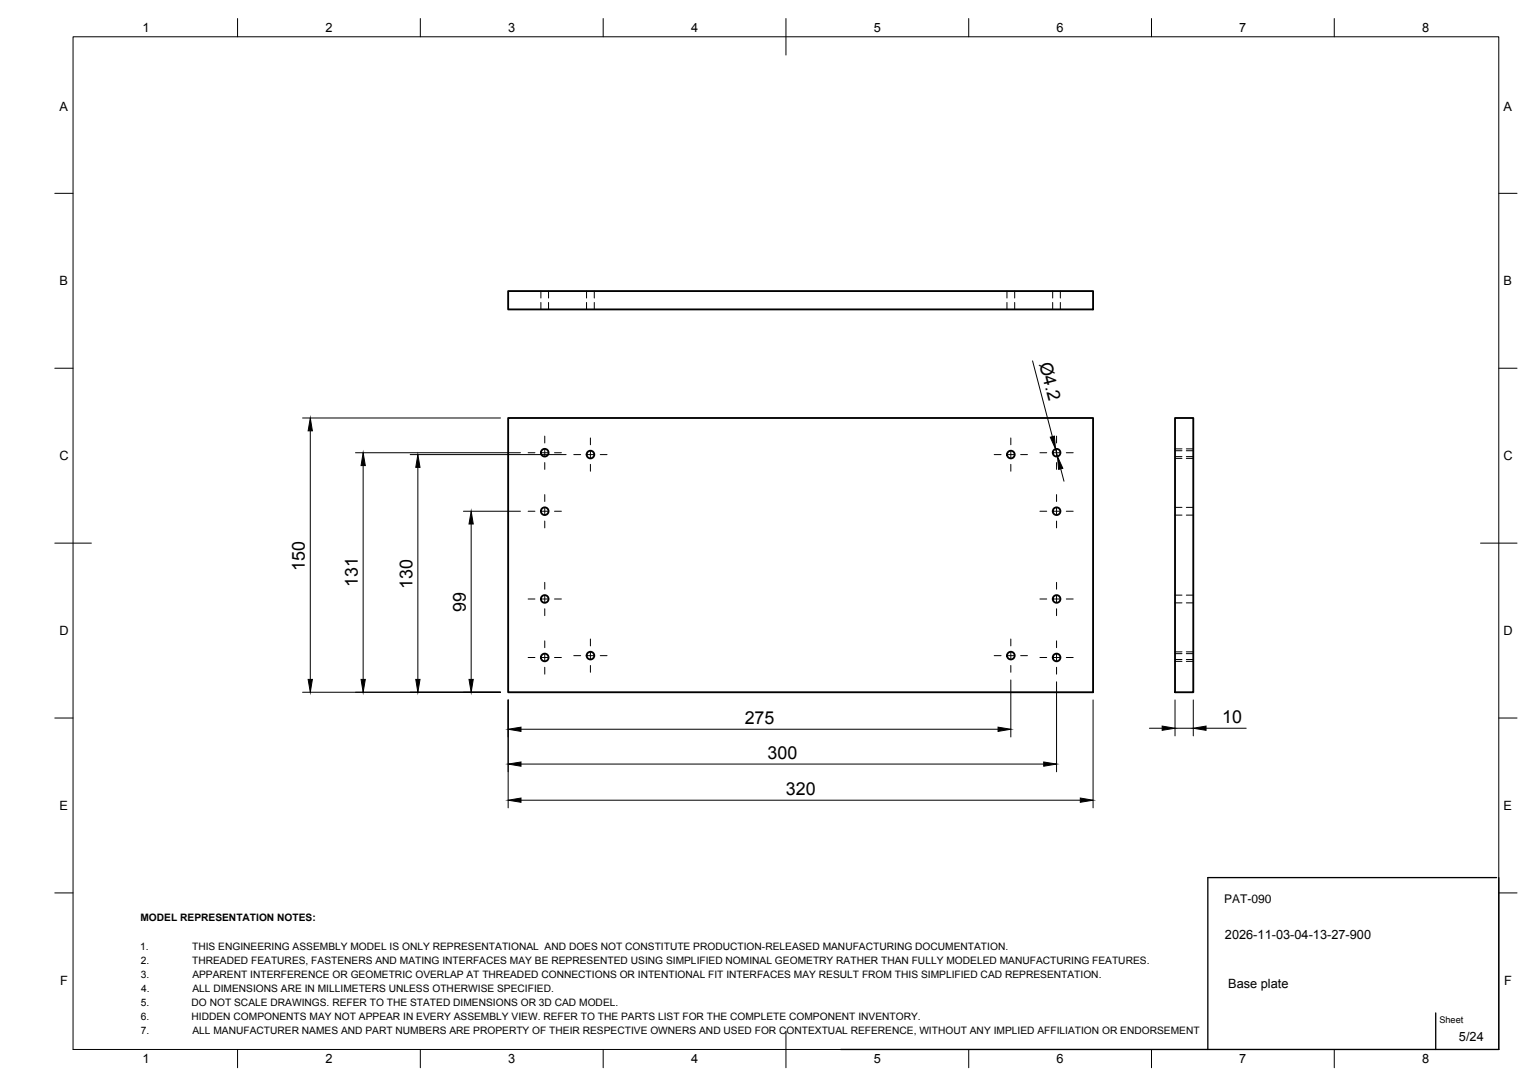
ISO-10303-21;
HEADER;
/* Generated by software containing ST-Developer
 * from STEP Tools, Inc. (www.steptools.com) 
 */

FILE_DESCRIPTION(
/* description */ ('Round-Shaft Linear Stage with Ball Bushings'),
/* implementation_level */ '2;1');

FILE_NAME(
/* name */ 'Base plate.step',
/* time_stamp */ '2026-10-27T10:47:55-07:00',
/* author */ (''),
/* organization */ (''),
/* preprocessor_version */ 'ST-DEVELOPER v20.2',
/* originating_system */ 'Autodesk Translation Framework v15.17.0.0',
/* authorisation */ '');

FILE_SCHEMA (('AUTOMOTIVE_DESIGN { 1 0 10303 214 3 1 1 }'));
ENDSEC;

DATA;
#10=MECHANICAL_DESIGN_GEOMETRIC_PRESENTATION_REPRESENTATION('',(#302),#7835);
#260=SHAPE_REPRESENTATION_RELATIONSHIP('SRR','None',#7948,#281);
#281=ADVANCED_BREP_SHAPE_REPRESENTATION('',(#323),#7812);
#302=STYLED_ITEM('',(#8123),#323);
#323=MANIFOLD_SOLID_BREP('Body1',#4392);
#340=FACE_BOUND('',#890,.T.);
#341=FACE_BOUND('',#891,.T.);
#342=FACE_BOUND('',#892,.T.);
#343=FACE_BOUND('',#893,.T.);
#344=FACE_BOUND('',#894,.T.);
#345=FACE_BOUND('',#895,.T.);
#346=FACE_BOUND('',#896,.T.);
#347=FACE_BOUND('',#897,.T.);
#348=FACE_BOUND('',#898,.T.);
#349=FACE_BOUND('',#899,.T.);
#350=FACE_BOUND('',#900,.T.);
#351=FACE_BOUND('',#901,.T.);
#352=FACE_BOUND('',#903,.T.);
#353=FACE_BOUND('',#904,.T.);
#354=FACE_BOUND('',#905,.T.);
#355=FACE_BOUND('',#906,.T.);
#356=FACE_BOUND('',#907,.T.);
#357=FACE_BOUND('',#908,.T.);
#358=FACE_BOUND('',#909,.T.);
#359=FACE_BOUND('',#910,.T.);
#360=FACE_BOUND('',#911,.T.);
#361=FACE_BOUND('',#912,.T.);
#362=FACE_BOUND('',#913,.T.);
#363=FACE_BOUND('',#914,.T.);
#459=PLANE('',#4688);
#460=PLANE('',#4689);
#461=PLANE('',#4690);
#462=PLANE('',#4691);
#463=PLANE('',#4692);
#464=PLANE('',#4693);
#616=FACE_OUTER_BOUND('',#873,.T.);
#617=FACE_OUTER_BOUND('',#874,.T.);
#618=FACE_OUTER_BOUND('',#875,.T.);
#619=FACE_OUTER_BOUND('',#876,.T.);
#620=FACE_OUTER_BOUND('',#877,.T.);
#621=FACE_OUTER_BOUND('',#878,.T.);
#622=FACE_OUTER_BOUND('',#879,.T.);
#623=FACE_OUTER_BOUND('',#880,.T.);
#624=FACE_OUTER_BOUND('',#881,.T.);
#625=FACE_OUTER_BOUND('',#882,.T.);
#626=FACE_OUTER_BOUND('',#883,.T.);
#627=FACE_OUTER_BOUND('',#884,.T.);
#628=FACE_OUTER_BOUND('',#885,.T.);
#629=FACE_OUTER_BOUND('',#886,.T.);
#630=FACE_OUTER_BOUND('',#887,.T.);
#631=FACE_OUTER_BOUND('',#888,.T.);
#632=FACE_OUTER_BOUND('',#889,.T.);
#633=FACE_OUTER_BOUND('',#902,.T.);
#873=EDGE_LOOP('',(#2994,#2995,#2996,#2997));
#874=EDGE_LOOP('',(#2998,#2999,#3000,#3001));
#875=EDGE_LOOP('',(#3002,#3003,#3004,#3005));
#876=EDGE_LOOP('',(#3006,#3007,#3008,#3009));
#877=EDGE_LOOP('',(#3010,#3011,#3012,#3013));
#878=EDGE_LOOP('',(#3014,#3015,#3016,#3017));
#879=EDGE_LOOP('',(#3018,#3019,#3020,#3021));
#880=EDGE_LOOP('',(#3022,#3023,#3024,#3025));
#881=EDGE_LOOP('',(#3026,#3027,#3028,#3029));
#882=EDGE_LOOP('',(#3030,#3031,#3032,#3033));
#883=EDGE_LOOP('',(#3034,#3035,#3036,#3037));
#884=EDGE_LOOP('',(#3038,#3039,#3040,#3041));
#885=EDGE_LOOP('',(#3042,#3043,#3044,#3045));
#886=EDGE_LOOP('',(#3046,#3047,#3048,#3049));
#887=EDGE_LOOP('',(#3050,#3051,#3052,#3053));
#888=EDGE_LOOP('',(#3054,#3055,#3056,#3057));
#889=EDGE_LOOP('',(#3058,#3059,#3060,#3061));
#890=EDGE_LOOP('',(#3062));
#891=EDGE_LOOP('',(#3063));
#892=EDGE_LOOP('',(#3064));
#893=EDGE_LOOP('',(#3065));
#894=EDGE_LOOP('',(#3066));
#895=EDGE_LOOP('',(#3067));
#896=EDGE_LOOP('',(#3068));
#897=EDGE_LOOP('',(#3069));
#898=EDGE_LOOP('',(#3070));
#899=EDGE_LOOP('',(#3071));
#900=EDGE_LOOP('',(#3072));
#901=EDGE_LOOP('',(#3073));
#902=EDGE_LOOP('',(#3074,#3075,#3076,#3077));
#903=EDGE_LOOP('',(#3078));
#904=EDGE_LOOP('',(#3079));
#905=EDGE_LOOP('',(#3080));
#906=EDGE_LOOP('',(#3081));
#907=EDGE_LOOP('',(#3082));
#908=EDGE_LOOP('',(#3083));
#909=EDGE_LOOP('',(#3084));
#910=EDGE_LOOP('',(#3085));
#911=EDGE_LOOP('',(#3086));
#912=EDGE_LOOP('',(#3087));
#913=EDGE_LOOP('',(#3088));
#914=EDGE_LOOP('',(#3089));
#1249=LINE('',#6577,#1589);
#1250=LINE('',#6583,#1590);
#1251=LINE('',#6589,#1591);
#1252=LINE('',#6595,#1592);
#1253=LINE('',#6601,#1593);
#1254=LINE('',#6607,#1594);
#1255=LINE('',#6613,#1595);
#1256=LINE('',#6619,#1596);
#1257=LINE('',#6625,#1597);
#1258=LINE('',#6631,#1598);
#1259=LINE('',#6637,#1599);
#1260=LINE('',#6643,#1600);
#1261=LINE('',#6648,#1601);
#1262=LINE('',#6650,#1602);
#1263=LINE('',#6652,#1603);
#1264=LINE('',#6653,#1604);
#1265=LINE('',#6656,#1605);
#1266=LINE('',#6658,#1606);
#1267=LINE('',#6659,#1607);
#1268=LINE('',#6662,#1608);
#1269=LINE('',#6664,#1609);
#1270=LINE('',#6665,#1610);
#1271=LINE('',#6667,#1611);
#1272=LINE('',#6668,#1612);
#1589=VECTOR('',#5186,0.210000000000001);
#1590=VECTOR('',#5193,0.21);
#1591=VECTOR('',#5200,0.21);
#1592=VECTOR('',#5207,0.210000000000001);
#1593=VECTOR('',#5214,0.210000000000001);
#1594=VECTOR('',#5221,0.210000000000001);
#1595=VECTOR('',#5228,0.21);
#1596=VECTOR('',#5235,0.21);
#1597=VECTOR('',#5242,0.21);
#1598=VECTOR('',#5249,0.21);
#1599=VECTOR('',#5256,0.210000000000001);
#1600=VECTOR('',#5263,0.210000000000001);
#1601=VECTOR('',#5268,1.);
#1602=VECTOR('',#5269,1.);
#1603=VECTOR('',#5270,1.);
#1604=VECTOR('',#5271,1.);
#1605=VECTOR('',#5274,1.);
#1606=VECTOR('',#5275,1.);
#1607=VECTOR('',#5276,1.);
#1608=VECTOR('',#5279,1.);
#1609=VECTOR('',#5280,1.);
#1610=VECTOR('',#5281,1.);
#1611=VECTOR('',#5284,1.);
#1612=VECTOR('',#5285,1.);
#1929=CIRCLE('',#4653,0.210000000000001);
#1930=CIRCLE('',#4654,0.210000000000001);
#1931=CIRCLE('',#4656,0.21);
#1932=CIRCLE('',#4657,0.21);
#1933=CIRCLE('',#4659,0.21);
#1934=CIRCLE('',#4660,0.21);
#1935=CIRCLE('',#4662,0.210000000000001);
#1936=CIRCLE('',#4663,0.210000000000001);
#1937=CIRCLE('',#4665,0.210000000000001);
#1938=CIRCLE('',#4666,0.210000000000001);
#1939=CIRCLE('',#4668,0.210000000000001);
#1940=CIRCLE('',#4669,0.210000000000001);
#1941=CIRCLE('',#4671,0.21);
#1942=CIRCLE('',#4672,0.21);
#1943=CIRCLE('',#4674,0.21);
#1944=CIRCLE('',#4675,0.21);
#1945=CIRCLE('',#4677,0.21);
#1946=CIRCLE('',#4678,0.21);
#1947=CIRCLE('',#4680,0.21);
#1948=CIRCLE('',#4681,0.21);
#1949=CIRCLE('',#4683,0.210000000000001);
#1950=CIRCLE('',#4684,0.210000000000001);
#1951=CIRCLE('',#4686,0.210000000000001);
#1952=CIRCLE('',#4687,0.210000000000001);
#2118=VERTEX_POINT('',#6574);
#2119=VERTEX_POINT('',#6576);
#2120=VERTEX_POINT('',#6580);
#2121=VERTEX_POINT('',#6582);
#2122=VERTEX_POINT('',#6586);
#2123=VERTEX_POINT('',#6588);
#2124=VERTEX_POINT('',#6592);
#2125=VERTEX_POINT('',#6594);
#2126=VERTEX_POINT('',#6598);
#2127=VERTEX_POINT('',#6600);
#2128=VERTEX_POINT('',#6604);
#2129=VERTEX_POINT('',#6606);
#2130=VERTEX_POINT('',#6610);
#2131=VERTEX_POINT('',#6612);
#2132=VERTEX_POINT('',#6616);
#2133=VERTEX_POINT('',#6618);
#2134=VERTEX_POINT('',#6622);
#2135=VERTEX_POINT('',#6624);
#2136=VERTEX_POINT('',#6628);
#2137=VERTEX_POINT('',#6630);
#2138=VERTEX_POINT('',#6634);
#2139=VERTEX_POINT('',#6636);
#2140=VERTEX_POINT('',#6640);
#2141=VERTEX_POINT('',#6642);
#2142=VERTEX_POINT('',#6646);
#2143=VERTEX_POINT('',#6647);
#2144=VERTEX_POINT('',#6649);
#2145=VERTEX_POINT('',#6651);
#2146=VERTEX_POINT('',#6655);
#2147=VERTEX_POINT('',#6657);
#2148=VERTEX_POINT('',#6661);
#2149=VERTEX_POINT('',#6663);
#2465=EDGE_CURVE('',#2118,#2118,#1929,.T.);
#2466=EDGE_CURVE('',#2118,#2119,#1249,.T.);
#2467=EDGE_CURVE('',#2119,#2119,#1930,.T.);
#2468=EDGE_CURVE('',#2120,#2120,#1931,.T.);
#2469=EDGE_CURVE('',#2120,#2121,#1250,.T.);
#2470=EDGE_CURVE('',#2121,#2121,#1932,.T.);
#2471=EDGE_CURVE('',#2122,#2122,#1933,.T.);
#2472=EDGE_CURVE('',#2122,#2123,#1251,.T.);
#2473=EDGE_CURVE('',#2123,#2123,#1934,.T.);
#2474=EDGE_CURVE('',#2124,#2124,#1935,.T.);
#2475=EDGE_CURVE('',#2124,#2125,#1252,.T.);
#2476=EDGE_CURVE('',#2125,#2125,#1936,.T.);
#2477=EDGE_CURVE('',#2126,#2126,#1937,.T.);
#2478=EDGE_CURVE('',#2126,#2127,#1253,.T.);
#2479=EDGE_CURVE('',#2127,#2127,#1938,.T.);
#2480=EDGE_CURVE('',#2128,#2128,#1939,.T.);
#2481=EDGE_CURVE('',#2128,#2129,#1254,.T.);
#2482=EDGE_CURVE('',#2129,#2129,#1940,.T.);
#2483=EDGE_CURVE('',#2130,#2130,#1941,.T.);
#2484=EDGE_CURVE('',#2130,#2131,#1255,.T.);
#2485=EDGE_CURVE('',#2131,#2131,#1942,.T.);
#2486=EDGE_CURVE('',#2132,#2132,#1943,.T.);
#2487=EDGE_CURVE('',#2132,#2133,#1256,.T.);
#2488=EDGE_CURVE('',#2133,#2133,#1944,.T.);
#2489=EDGE_CURVE('',#2134,#2134,#1945,.T.);
#2490=EDGE_CURVE('',#2134,#2135,#1257,.T.);
#2491=EDGE_CURVE('',#2135,#2135,#1946,.T.);
#2492=EDGE_CURVE('',#2136,#2136,#1947,.T.);
#2493=EDGE_CURVE('',#2136,#2137,#1258,.T.);
#2494=EDGE_CURVE('',#2137,#2137,#1948,.T.);
#2495=EDGE_CURVE('',#2138,#2138,#1949,.T.);
#2496=EDGE_CURVE('',#2138,#2139,#1259,.T.);
#2497=EDGE_CURVE('',#2139,#2139,#1950,.T.);
#2498=EDGE_CURVE('',#2140,#2140,#1951,.T.);
#2499=EDGE_CURVE('',#2140,#2141,#1260,.T.);
#2500=EDGE_CURVE('',#2141,#2141,#1952,.T.);
#2501=EDGE_CURVE('',#2142,#2143,#1261,.T.);
#2502=EDGE_CURVE('',#2143,#2144,#1262,.T.);
#2503=EDGE_CURVE('',#2145,#2144,#1263,.T.);
#2504=EDGE_CURVE('',#2142,#2145,#1264,.T.);
#2505=EDGE_CURVE('',#2146,#2142,#1265,.T.);
#2506=EDGE_CURVE('',#2147,#2145,#1266,.T.);
#2507=EDGE_CURVE('',#2146,#2147,#1267,.T.);
#2508=EDGE_CURVE('',#2148,#2146,#1268,.T.);
#2509=EDGE_CURVE('',#2149,#2147,#1269,.T.);
#2510=EDGE_CURVE('',#2148,#2149,#1270,.T.);
#2511=EDGE_CURVE('',#2143,#2148,#1271,.T.);
#2512=EDGE_CURVE('',#2144,#2149,#1272,.T.);
#2994=ORIENTED_EDGE('',*,*,#2465,.F.);
#2995=ORIENTED_EDGE('',*,*,#2466,.T.);
#2996=ORIENTED_EDGE('',*,*,#2467,.F.);
#2997=ORIENTED_EDGE('',*,*,#2466,.F.);
#2998=ORIENTED_EDGE('',*,*,#2468,.F.);
#2999=ORIENTED_EDGE('',*,*,#2469,.T.);
#3000=ORIENTED_EDGE('',*,*,#2470,.F.);
#3001=ORIENTED_EDGE('',*,*,#2469,.F.);
#3002=ORIENTED_EDGE('',*,*,#2471,.F.);
#3003=ORIENTED_EDGE('',*,*,#2472,.T.);
#3004=ORIENTED_EDGE('',*,*,#2473,.F.);
#3005=ORIENTED_EDGE('',*,*,#2472,.F.);
#3006=ORIENTED_EDGE('',*,*,#2474,.F.);
#3007=ORIENTED_EDGE('',*,*,#2475,.T.);
#3008=ORIENTED_EDGE('',*,*,#2476,.F.);
#3009=ORIENTED_EDGE('',*,*,#2475,.F.);
#3010=ORIENTED_EDGE('',*,*,#2477,.F.);
#3011=ORIENTED_EDGE('',*,*,#2478,.T.);
#3012=ORIENTED_EDGE('',*,*,#2479,.F.);
#3013=ORIENTED_EDGE('',*,*,#2478,.F.);
#3014=ORIENTED_EDGE('',*,*,#2480,.F.);
#3015=ORIENTED_EDGE('',*,*,#2481,.T.);
#3016=ORIENTED_EDGE('',*,*,#2482,.F.);
#3017=ORIENTED_EDGE('',*,*,#2481,.F.);
#3018=ORIENTED_EDGE('',*,*,#2483,.F.);
#3019=ORIENTED_EDGE('',*,*,#2484,.T.);
#3020=ORIENTED_EDGE('',*,*,#2485,.F.);
#3021=ORIENTED_EDGE('',*,*,#2484,.F.);
#3022=ORIENTED_EDGE('',*,*,#2486,.F.);
#3023=ORIENTED_EDGE('',*,*,#2487,.T.);
#3024=ORIENTED_EDGE('',*,*,#2488,.F.);
#3025=ORIENTED_EDGE('',*,*,#2487,.F.);
#3026=ORIENTED_EDGE('',*,*,#2489,.F.);
#3027=ORIENTED_EDGE('',*,*,#2490,.T.);
#3028=ORIENTED_EDGE('',*,*,#2491,.F.);
#3029=ORIENTED_EDGE('',*,*,#2490,.F.);
#3030=ORIENTED_EDGE('',*,*,#2492,.F.);
#3031=ORIENTED_EDGE('',*,*,#2493,.T.);
#3032=ORIENTED_EDGE('',*,*,#2494,.F.);
#3033=ORIENTED_EDGE('',*,*,#2493,.F.);
#3034=ORIENTED_EDGE('',*,*,#2495,.F.);
#3035=ORIENTED_EDGE('',*,*,#2496,.T.);
#3036=ORIENTED_EDGE('',*,*,#2497,.F.);
#3037=ORIENTED_EDGE('',*,*,#2496,.F.);
#3038=ORIENTED_EDGE('',*,*,#2498,.F.);
#3039=ORIENTED_EDGE('',*,*,#2499,.T.);
#3040=ORIENTED_EDGE('',*,*,#2500,.F.);
#3041=ORIENTED_EDGE('',*,*,#2499,.F.);
#3042=ORIENTED_EDGE('',*,*,#2501,.T.);
#3043=ORIENTED_EDGE('',*,*,#2502,.T.);
#3044=ORIENTED_EDGE('',*,*,#2503,.F.);
#3045=ORIENTED_EDGE('',*,*,#2504,.F.);
#3046=ORIENTED_EDGE('',*,*,#2505,.T.);
#3047=ORIENTED_EDGE('',*,*,#2504,.T.);
#3048=ORIENTED_EDGE('',*,*,#2506,.F.);
#3049=ORIENTED_EDGE('',*,*,#2507,.F.);
#3050=ORIENTED_EDGE('',*,*,#2508,.T.);
#3051=ORIENTED_EDGE('',*,*,#2507,.T.);
#3052=ORIENTED_EDGE('',*,*,#2509,.F.);
#3053=ORIENTED_EDGE('',*,*,#2510,.F.);
#3054=ORIENTED_EDGE('',*,*,#2511,.T.);
#3055=ORIENTED_EDGE('',*,*,#2510,.T.);
#3056=ORIENTED_EDGE('',*,*,#2512,.F.);
#3057=ORIENTED_EDGE('',*,*,#2502,.F.);
#3058=ORIENTED_EDGE('',*,*,#2512,.T.);
#3059=ORIENTED_EDGE('',*,*,#2509,.T.);
#3060=ORIENTED_EDGE('',*,*,#2506,.T.);
#3061=ORIENTED_EDGE('',*,*,#2503,.T.);
#3062=ORIENTED_EDGE('',*,*,#2479,.T.);
#3063=ORIENTED_EDGE('',*,*,#2482,.T.);
#3064=ORIENTED_EDGE('',*,*,#2485,.T.);
#3065=ORIENTED_EDGE('',*,*,#2488,.T.);
#3066=ORIENTED_EDGE('',*,*,#2491,.T.);
#3067=ORIENTED_EDGE('',*,*,#2494,.T.);
#3068=ORIENTED_EDGE('',*,*,#2497,.T.);
#3069=ORIENTED_EDGE('',*,*,#2500,.T.);
#3070=ORIENTED_EDGE('',*,*,#2476,.T.);
#3071=ORIENTED_EDGE('',*,*,#2473,.T.);
#3072=ORIENTED_EDGE('',*,*,#2470,.T.);
#3073=ORIENTED_EDGE('',*,*,#2467,.T.);
#3074=ORIENTED_EDGE('',*,*,#2511,.F.);
#3075=ORIENTED_EDGE('',*,*,#2501,.F.);
#3076=ORIENTED_EDGE('',*,*,#2505,.F.);
#3077=ORIENTED_EDGE('',*,*,#2508,.F.);
#3078=ORIENTED_EDGE('',*,*,#2477,.T.);
#3079=ORIENTED_EDGE('',*,*,#2480,.T.);
#3080=ORIENTED_EDGE('',*,*,#2483,.T.);
#3081=ORIENTED_EDGE('',*,*,#2486,.T.);
#3082=ORIENTED_EDGE('',*,*,#2489,.T.);
#3083=ORIENTED_EDGE('',*,*,#2492,.T.);
#3084=ORIENTED_EDGE('',*,*,#2495,.T.);
#3085=ORIENTED_EDGE('',*,*,#2498,.T.);
#3086=ORIENTED_EDGE('',*,*,#2474,.T.);
#3087=ORIENTED_EDGE('',*,*,#2471,.T.);
#3088=ORIENTED_EDGE('',*,*,#2468,.T.);
#3089=ORIENTED_EDGE('',*,*,#2465,.T.);
#4052=CYLINDRICAL_SURFACE('',#4652,0.210000000000001);
#4053=CYLINDRICAL_SURFACE('',#4655,0.21);
#4054=CYLINDRICAL_SURFACE('',#4658,0.21);
#4055=CYLINDRICAL_SURFACE('',#4661,0.210000000000001);
#4056=CYLINDRICAL_SURFACE('',#4664,0.210000000000001);
#4057=CYLINDRICAL_SURFACE('',#4667,0.210000000000001);
#4058=CYLINDRICAL_SURFACE('',#4670,0.21);
#4059=CYLINDRICAL_SURFACE('',#4673,0.21);
#4060=CYLINDRICAL_SURFACE('',#4676,0.21);
#4061=CYLINDRICAL_SURFACE('',#4679,0.21);
#4062=CYLINDRICAL_SURFACE('',#4682,0.210000000000001);
#4063=CYLINDRICAL_SURFACE('',#4685,0.210000000000001);
#4135=ADVANCED_FACE('',(#616),#4052,.F.);
#4136=ADVANCED_FACE('',(#617),#4053,.F.);
#4137=ADVANCED_FACE('',(#618),#4054,.F.);
#4138=ADVANCED_FACE('',(#619),#4055,.F.);
#4139=ADVANCED_FACE('',(#620),#4056,.F.);
#4140=ADVANCED_FACE('',(#621),#4057,.F.);
#4141=ADVANCED_FACE('',(#622),#4058,.F.);
#4142=ADVANCED_FACE('',(#623),#4059,.F.);
#4143=ADVANCED_FACE('',(#624),#4060,.F.);
#4144=ADVANCED_FACE('',(#625),#4061,.F.);
#4145=ADVANCED_FACE('',(#626),#4062,.F.);
#4146=ADVANCED_FACE('',(#627),#4063,.F.);
#4147=ADVANCED_FACE('',(#628),#459,.T.);
#4148=ADVANCED_FACE('',(#629),#460,.T.);
#4149=ADVANCED_FACE('',(#630),#461,.T.);
#4150=ADVANCED_FACE('',(#631),#462,.T.);
#4151=ADVANCED_FACE('',(#632,#340,#341,#342,#343,#344,#345,#346,#347,#348,
#349,#350,#351),#463,.T.);
#4152=ADVANCED_FACE('',(#633,#352,#353,#354,#355,#356,#357,#358,#359,#360,
#361,#362,#363),#464,.F.);
#4392=CLOSED_SHELL('',(#4135,#4136,#4137,#4138,#4139,#4140,#4141,#4142,
#4143,#4144,#4145,#4146,#4147,#4148,#4149,#4150,#4151,#4152));
#4651=AXIS2_PLACEMENT_3D('',#6572,#5180,#5181);
#4652=AXIS2_PLACEMENT_3D('',#6573,#5182,#5183);
#4653=AXIS2_PLACEMENT_3D('',#6575,#5184,#5185);
#4654=AXIS2_PLACEMENT_3D('',#6578,#5187,#5188);
#4655=AXIS2_PLACEMENT_3D('',#6579,#5189,#5190);
#4656=AXIS2_PLACEMENT_3D('',#6581,#5191,#5192);
#4657=AXIS2_PLACEMENT_3D('',#6584,#5194,#5195);
#4658=AXIS2_PLACEMENT_3D('',#6585,#5196,#5197);
#4659=AXIS2_PLACEMENT_3D('',#6587,#5198,#5199);
#4660=AXIS2_PLACEMENT_3D('',#6590,#5201,#5202);
#4661=AXIS2_PLACEMENT_3D('',#6591,#5203,#5204);
#4662=AXIS2_PLACEMENT_3D('',#6593,#5205,#5206);
#4663=AXIS2_PLACEMENT_3D('',#6596,#5208,#5209);
#4664=AXIS2_PLACEMENT_3D('',#6597,#5210,#5211);
#4665=AXIS2_PLACEMENT_3D('',#6599,#5212,#5213);
#4666=AXIS2_PLACEMENT_3D('',#6602,#5215,#5216);
#4667=AXIS2_PLACEMENT_3D('',#6603,#5217,#5218);
#4668=AXIS2_PLACEMENT_3D('',#6605,#5219,#5220);
#4669=AXIS2_PLACEMENT_3D('',#6608,#5222,#5223);
#4670=AXIS2_PLACEMENT_3D('',#6609,#5224,#5225);
#4671=AXIS2_PLACEMENT_3D('',#6611,#5226,#5227);
#4672=AXIS2_PLACEMENT_3D('',#6614,#5229,#5230);
#4673=AXIS2_PLACEMENT_3D('',#6615,#5231,#5232);
#4674=AXIS2_PLACEMENT_3D('',#6617,#5233,#5234);
#4675=AXIS2_PLACEMENT_3D('',#6620,#5236,#5237);
#4676=AXIS2_PLACEMENT_3D('',#6621,#5238,#5239);
#4677=AXIS2_PLACEMENT_3D('',#6623,#5240,#5241);
#4678=AXIS2_PLACEMENT_3D('',#6626,#5243,#5244);
#4679=AXIS2_PLACEMENT_3D('',#6627,#5245,#5246);
#4680=AXIS2_PLACEMENT_3D('',#6629,#5247,#5248);
#4681=AXIS2_PLACEMENT_3D('',#6632,#5250,#5251);
#4682=AXIS2_PLACEMENT_3D('',#6633,#5252,#5253);
#4683=AXIS2_PLACEMENT_3D('',#6635,#5254,#5255);
#4684=AXIS2_PLACEMENT_3D('',#6638,#5257,#5258);
#4685=AXIS2_PLACEMENT_3D('',#6639,#5259,#5260);
#4686=AXIS2_PLACEMENT_3D('',#6641,#5261,#5262);
#4687=AXIS2_PLACEMENT_3D('',#6644,#5264,#5265);
#4688=AXIS2_PLACEMENT_3D('',#6645,#5266,#5267);
#4689=AXIS2_PLACEMENT_3D('',#6654,#5272,#5273);
#4690=AXIS2_PLACEMENT_3D('',#6660,#5277,#5278);
#4691=AXIS2_PLACEMENT_3D('',#6666,#5282,#5283);
#4692=AXIS2_PLACEMENT_3D('',#6669,#5286,#5287);
#4693=AXIS2_PLACEMENT_3D('',#6670,#5288,#5289);
#5180=DIRECTION('axis',(0.,0.,1.));
#5181=DIRECTION('refdir',(1.,0.,0.));
#5182=DIRECTION('center_axis',(0.,0.,1.));
#5183=DIRECTION('ref_axis',(1.,0.,0.));
#5184=DIRECTION('center_axis',(0.,0.,1.));
#5185=DIRECTION('ref_axis',(1.,0.,0.));
#5186=DIRECTION('',(0.,0.,1.));
#5187=DIRECTION('center_axis',(0.,0.,-1.));
#5188=DIRECTION('ref_axis',(1.,0.,0.));
#5189=DIRECTION('center_axis',(0.,0.,1.));
#5190=DIRECTION('ref_axis',(1.,0.,0.));
#5191=DIRECTION('center_axis',(0.,0.,1.));
#5192=DIRECTION('ref_axis',(1.,0.,0.));
#5193=DIRECTION('',(0.,0.,1.));
#5194=DIRECTION('center_axis',(0.,0.,-1.));
#5195=DIRECTION('ref_axis',(1.,0.,0.));
#5196=DIRECTION('center_axis',(0.,0.,1.));
#5197=DIRECTION('ref_axis',(1.,0.,0.));
#5198=DIRECTION('center_axis',(0.,0.,1.));
#5199=DIRECTION('ref_axis',(1.,0.,0.));
#5200=DIRECTION('',(0.,0.,1.));
#5201=DIRECTION('center_axis',(0.,0.,-1.));
#5202=DIRECTION('ref_axis',(1.,0.,0.));
#5203=DIRECTION('center_axis',(0.,0.,1.));
#5204=DIRECTION('ref_axis',(1.,0.,0.));
#5205=DIRECTION('center_axis',(0.,0.,1.));
#5206=DIRECTION('ref_axis',(1.,0.,0.));
#5207=DIRECTION('',(0.,0.,1.));
#5208=DIRECTION('center_axis',(0.,0.,-1.));
#5209=DIRECTION('ref_axis',(1.,0.,0.));
#5210=DIRECTION('center_axis',(0.,0.,1.));
#5211=DIRECTION('ref_axis',(1.,0.,0.));
#5212=DIRECTION('center_axis',(0.,0.,1.));
#5213=DIRECTION('ref_axis',(1.,0.,0.));
#5214=DIRECTION('',(0.,0.,1.));
#5215=DIRECTION('center_axis',(0.,0.,-1.));
#5216=DIRECTION('ref_axis',(1.,0.,0.));
#5217=DIRECTION('center_axis',(0.,0.,1.));
#5218=DIRECTION('ref_axis',(1.,0.,0.));
#5219=DIRECTION('center_axis',(0.,0.,1.));
#5220=DIRECTION('ref_axis',(1.,0.,0.));
#5221=DIRECTION('',(0.,0.,1.));
#5222=DIRECTION('center_axis',(0.,0.,-1.));
#5223=DIRECTION('ref_axis',(1.,0.,0.));
#5224=DIRECTION('center_axis',(0.,0.,1.));
#5225=DIRECTION('ref_axis',(1.,0.,0.));
#5226=DIRECTION('center_axis',(0.,0.,1.));
#5227=DIRECTION('ref_axis',(1.,0.,0.));
#5228=DIRECTION('',(0.,0.,1.));
#5229=DIRECTION('center_axis',(0.,0.,-1.));
#5230=DIRECTION('ref_axis',(1.,0.,0.));
#5231=DIRECTION('center_axis',(0.,0.,1.));
#5232=DIRECTION('ref_axis',(1.,0.,0.));
#5233=DIRECTION('center_axis',(0.,0.,1.));
#5234=DIRECTION('ref_axis',(1.,0.,0.));
#5235=DIRECTION('',(0.,0.,1.));
#5236=DIRECTION('center_axis',(0.,0.,-1.));
#5237=DIRECTION('ref_axis',(1.,0.,0.));
#5238=DIRECTION('center_axis',(0.,0.,1.));
#5239=DIRECTION('ref_axis',(1.,0.,0.));
#5240=DIRECTION('center_axis',(0.,0.,1.));
#5241=DIRECTION('ref_axis',(1.,0.,0.));
#5242=DIRECTION('',(0.,0.,1.));
#5243=DIRECTION('center_axis',(0.,0.,-1.));
#5244=DIRECTION('ref_axis',(1.,0.,0.));
#5245=DIRECTION('center_axis',(0.,0.,1.));
#5246=DIRECTION('ref_axis',(1.,0.,0.));
#5247=DIRECTION('center_axis',(0.,0.,1.));
#5248=DIRECTION('ref_axis',(1.,0.,0.));
#5249=DIRECTION('',(0.,0.,1.));
#5250=DIRECTION('center_axis',(0.,0.,-1.));
#5251=DIRECTION('ref_axis',(1.,0.,0.));
#5252=DIRECTION('center_axis',(0.,0.,1.));
#5253=DIRECTION('ref_axis',(1.,0.,0.));
#5254=DIRECTION('center_axis',(0.,0.,1.));
#5255=DIRECTION('ref_axis',(1.,0.,0.));
#5256=DIRECTION('',(0.,0.,1.));
#5257=DIRECTION('center_axis',(0.,0.,-1.));
#5258=DIRECTION('ref_axis',(1.,0.,0.));
#5259=DIRECTION('center_axis',(0.,0.,1.));
#5260=DIRECTION('ref_axis',(1.,0.,0.));
#5261=DIRECTION('center_axis',(0.,0.,1.));
#5262=DIRECTION('ref_axis',(1.,0.,0.));
#5263=DIRECTION('',(0.,0.,1.));
#5264=DIRECTION('center_axis',(0.,0.,-1.));
#5265=DIRECTION('ref_axis',(1.,0.,0.));
#5266=DIRECTION('center_axis',(0.,1.,0.));
#5267=DIRECTION('ref_axis',(-1.,0.,0.));
#5268=DIRECTION('',(-1.,0.,0.));
#5269=DIRECTION('',(0.,0.,1.));
#5270=DIRECTION('',(-1.,0.,0.));
#5271=DIRECTION('',(0.,0.,1.));
#5272=DIRECTION('center_axis',(1.,0.,0.));
#5273=DIRECTION('ref_axis',(0.,1.,0.));
#5274=DIRECTION('',(0.,1.,0.));
#5275=DIRECTION('',(0.,1.,0.));
#5276=DIRECTION('',(0.,0.,1.));
#5277=DIRECTION('center_axis',(0.,-1.,0.));
#5278=DIRECTION('ref_axis',(1.,0.,0.));
#5279=DIRECTION('',(1.,0.,0.));
#5280=DIRECTION('',(1.,0.,0.));
#5281=DIRECTION('',(0.,0.,1.));
#5282=DIRECTION('center_axis',(-1.,0.,0.));
#5283=DIRECTION('ref_axis',(0.,-1.,0.));
#5284=DIRECTION('',(0.,-1.,0.));
#5285=DIRECTION('',(0.,-1.,0.));
#5286=DIRECTION('center_axis',(0.,0.,1.));
#5287=DIRECTION('ref_axis',(1.,0.,0.));
#5288=DIRECTION('center_axis',(0.,0.,1.));
#5289=DIRECTION('ref_axis',(1.,0.,0.));
#6572=CARTESIAN_POINT('',(0.,0.,0.));
#6573=CARTESIAN_POINT('Origin',(26.5,-5.5,-0.1));
#6574=CARTESIAN_POINT('',(26.29,-5.5,0.));
#6575=CARTESIAN_POINT('Origin',(26.5,-5.5,0.));
#6576=CARTESIAN_POINT('',(26.29,-5.5,1.));
#6577=CARTESIAN_POINT('',(26.29,-5.5,-0.1));
#6578=CARTESIAN_POINT('Origin',(26.5,-5.5,1.));
#6579=CARTESIAN_POINT('Origin',(3.5,5.5,-0.1));
#6580=CARTESIAN_POINT('',(3.29,5.5,0.));
#6581=CARTESIAN_POINT('Origin',(3.5,5.5,0.));
#6582=CARTESIAN_POINT('',(3.29,5.5,1.));
#6583=CARTESIAN_POINT('',(3.29,5.5,-0.1));
#6584=CARTESIAN_POINT('Origin',(3.5,5.5,1.));
#6585=CARTESIAN_POINT('Origin',(3.5,-5.5,-0.1));
#6586=CARTESIAN_POINT('',(3.29,-5.5,0.));
#6587=CARTESIAN_POINT('Origin',(3.5,-5.5,0.));
#6588=CARTESIAN_POINT('',(3.29,-5.5,1.));
#6589=CARTESIAN_POINT('',(3.29,-5.5,-0.1));
#6590=CARTESIAN_POINT('Origin',(3.5,-5.5,1.));
#6591=CARTESIAN_POINT('Origin',(26.5,5.5,-0.1));
#6592=CARTESIAN_POINT('',(26.29,5.5,0.));
#6593=CARTESIAN_POINT('Origin',(26.5,5.5,0.));
#6594=CARTESIAN_POINT('',(26.29,5.5,1.));
#6595=CARTESIAN_POINT('',(26.29,5.5,-0.1));
#6596=CARTESIAN_POINT('Origin',(26.5,5.5,1.));
#6597=CARTESIAN_POINT('Origin',(29.,2.4,-0.1));
#6598=CARTESIAN_POINT('',(28.79,2.4,0.));
#6599=CARTESIAN_POINT('Origin',(29.,2.4,0.));
#6600=CARTESIAN_POINT('',(28.79,2.4,1.));
#6601=CARTESIAN_POINT('',(28.79,2.4,-0.1));
#6602=CARTESIAN_POINT('Origin',(29.,2.4,1.));
#6603=CARTESIAN_POINT('Origin',(29.,-5.6,-0.1));
#6604=CARTESIAN_POINT('',(28.79,-5.6,0.));
#6605=CARTESIAN_POINT('Origin',(29.,-5.6,0.));
#6606=CARTESIAN_POINT('',(28.79,-5.6,1.));
#6607=CARTESIAN_POINT('',(28.79,-5.6,-0.1));
#6608=CARTESIAN_POINT('Origin',(29.,-5.6,1.));
#6609=CARTESIAN_POINT('Origin',(1.,5.6,-0.1));
#6610=CARTESIAN_POINT('',(0.79,5.6,0.));
#6611=CARTESIAN_POINT('Origin',(1.,5.6,0.));
#6612=CARTESIAN_POINT('',(0.79,5.6,1.));
#6613=CARTESIAN_POINT('',(0.79,5.6,-0.1));
#6614=CARTESIAN_POINT('Origin',(1.,5.6,1.));
#6615=CARTESIAN_POINT('Origin',(1.,-2.4,-0.1));
#6616=CARTESIAN_POINT('',(0.79,-2.4,0.));
#6617=CARTESIAN_POINT('Origin',(1.,-2.4,0.));
#6618=CARTESIAN_POINT('',(0.79,-2.4,1.));
#6619=CARTESIAN_POINT('',(0.79,-2.4,-0.1));
#6620=CARTESIAN_POINT('Origin',(1.,-2.4,1.));
#6621=CARTESIAN_POINT('Origin',(1.,2.4,-0.1));
#6622=CARTESIAN_POINT('',(0.79,2.4,0.));
#6623=CARTESIAN_POINT('Origin',(1.,2.4,0.));
#6624=CARTESIAN_POINT('',(0.79,2.4,1.));
#6625=CARTESIAN_POINT('',(0.79,2.4,-0.1));
#6626=CARTESIAN_POINT('Origin',(1.,2.4,1.));
#6627=CARTESIAN_POINT('Origin',(1.,-5.6,-0.1));
#6628=CARTESIAN_POINT('',(0.79,-5.6,0.));
#6629=CARTESIAN_POINT('Origin',(1.,-5.6,0.));
#6630=CARTESIAN_POINT('',(0.79,-5.6,1.));
#6631=CARTESIAN_POINT('',(0.79,-5.6,-0.1));
#6632=CARTESIAN_POINT('Origin',(1.,-5.6,1.));
#6633=CARTESIAN_POINT('Origin',(29.,-2.4,-0.1));
#6634=CARTESIAN_POINT('',(28.79,-2.4,0.));
#6635=CARTESIAN_POINT('Origin',(29.,-2.4,0.));
#6636=CARTESIAN_POINT('',(28.79,-2.4,1.));
#6637=CARTESIAN_POINT('',(28.79,-2.4,-0.1));
#6638=CARTESIAN_POINT('Origin',(29.,-2.4,1.));
#6639=CARTESIAN_POINT('Origin',(29.,5.6,-0.1));
#6640=CARTESIAN_POINT('',(28.79,5.6,0.));
#6641=CARTESIAN_POINT('Origin',(29.,5.6,0.));
#6642=CARTESIAN_POINT('',(28.79,5.6,1.));
#6643=CARTESIAN_POINT('',(28.79,5.6,-0.1));
#6644=CARTESIAN_POINT('Origin',(29.,5.6,1.));
#6645=CARTESIAN_POINT('Origin',(31.,7.5,0.));
#6646=CARTESIAN_POINT('',(31.,7.5,0.));
#6647=CARTESIAN_POINT('',(-1.,7.5,0.));
#6648=CARTESIAN_POINT('',(31.,7.5,0.));
#6649=CARTESIAN_POINT('',(-1.,7.5,1.));
#6650=CARTESIAN_POINT('',(-1.,7.5,0.));
#6651=CARTESIAN_POINT('',(31.,7.5,1.));
#6652=CARTESIAN_POINT('',(31.,7.5,1.));
#6653=CARTESIAN_POINT('',(31.,7.5,0.));
#6654=CARTESIAN_POINT('Origin',(31.,-7.5,0.));
#6655=CARTESIAN_POINT('',(31.,-7.5,0.));
#6656=CARTESIAN_POINT('',(31.,-7.5,0.));
#6657=CARTESIAN_POINT('',(31.,-7.5,1.));
#6658=CARTESIAN_POINT('',(31.,-7.5,1.));
#6659=CARTESIAN_POINT('',(31.,-7.5,0.));
#6660=CARTESIAN_POINT('Origin',(-1.,-7.5,0.));
#6661=CARTESIAN_POINT('',(-1.,-7.5,0.));
#6662=CARTESIAN_POINT('',(-1.,-7.5,0.));
#6663=CARTESIAN_POINT('',(-1.,-7.5,1.));
#6664=CARTESIAN_POINT('',(-1.,-7.5,1.));
#6665=CARTESIAN_POINT('',(-1.,-7.5,0.));
#6666=CARTESIAN_POINT('Origin',(-1.,7.5,0.));
#6667=CARTESIAN_POINT('',(-1.,7.5,0.));
#6668=CARTESIAN_POINT('',(-1.,7.5,1.));
#6669=CARTESIAN_POINT('Origin',(15.,0.,1.));
#6670=CARTESIAN_POINT('Origin',(15.,0.,0.));
#7786=UNCERTAINTY_MEASURE_WITH_UNIT(LENGTH_MEASURE(0.001),#7836,
'DISTANCE_ACCURACY_VALUE',
'Maximum model space distance between geometric entities at asserted c
onnectivities');
#7809=UNCERTAINTY_MEASURE_WITH_UNIT(LENGTH_MEASURE(0.001),#7836,
'DISTANCE_ACCURACY_VALUE',
'Maximum model space distance between geometric entities at asserted c
onnectivities');
#7812=(
GEOMETRIC_REPRESENTATION_CONTEXT(3)
GLOBAL_UNCERTAINTY_ASSIGNED_CONTEXT((#7786))
GLOBAL_UNIT_ASSIGNED_CONTEXT((#7836,#7838,#7839))
REPRESENTATION_CONTEXT('','3D')
);
#7835=(
GEOMETRIC_REPRESENTATION_CONTEXT(3)
GLOBAL_UNCERTAINTY_ASSIGNED_CONTEXT((#7809))
GLOBAL_UNIT_ASSIGNED_CONTEXT((#7836,#7838,#7839))
REPRESENTATION_CONTEXT('','3D')
);
#7836=(
LENGTH_UNIT()
NAMED_UNIT(*)
SI_UNIT(.CENTI.,.METRE.)
);
#7838=(
NAMED_UNIT(*)
PLANE_ANGLE_UNIT()
SI_UNIT($,.RADIAN.)
);
#7839=(
NAMED_UNIT(*)
SI_UNIT($,.STERADIAN.)
SOLID_ANGLE_UNIT()
);
#7842=SHAPE_DEFINITION_REPRESENTATION(#7867,#7948);
#7867=PRODUCT_DEFINITION_SHAPE('',$,#7974);
#7948=SHAPE_REPRESENTATION('',(#4651),#7812);
#7971=PRODUCT_DEFINITION_CONTEXT('part definition',#8048,'design');
#7974=PRODUCT_DEFINITION('Base plate','Base plate',#7999,#7971);
#7999=PRODUCT_DEFINITION_FORMATION('',$,#8052);
#8048=APPLICATION_CONTEXT(
'Core Data for Automotive Mechanical Design Process');
#8049=PRODUCT_CONTEXT('part definition',#8048,'mechanical');
#8052=PRODUCT('Base plate','Base plate','Base plate',(#8049));
#8117=COLOUR_RGB('Dark Blue',0.08,0.2,0.34);
#8118=FILL_AREA_STYLE_COLOUR('',#8117);
#8119=FILL_AREA_STYLE('',(#8118));
#8120=SURFACE_STYLE_FILL_AREA(#8119);
#8121=SURFACE_SIDE_STYLE('',(#8120));
#8122=SURFACE_STYLE_USAGE(.BOTH.,#8121);
#8123=PRESENTATION_STYLE_ASSIGNMENT((#8122));
ENDSEC;
END-ISO-10303-21;
